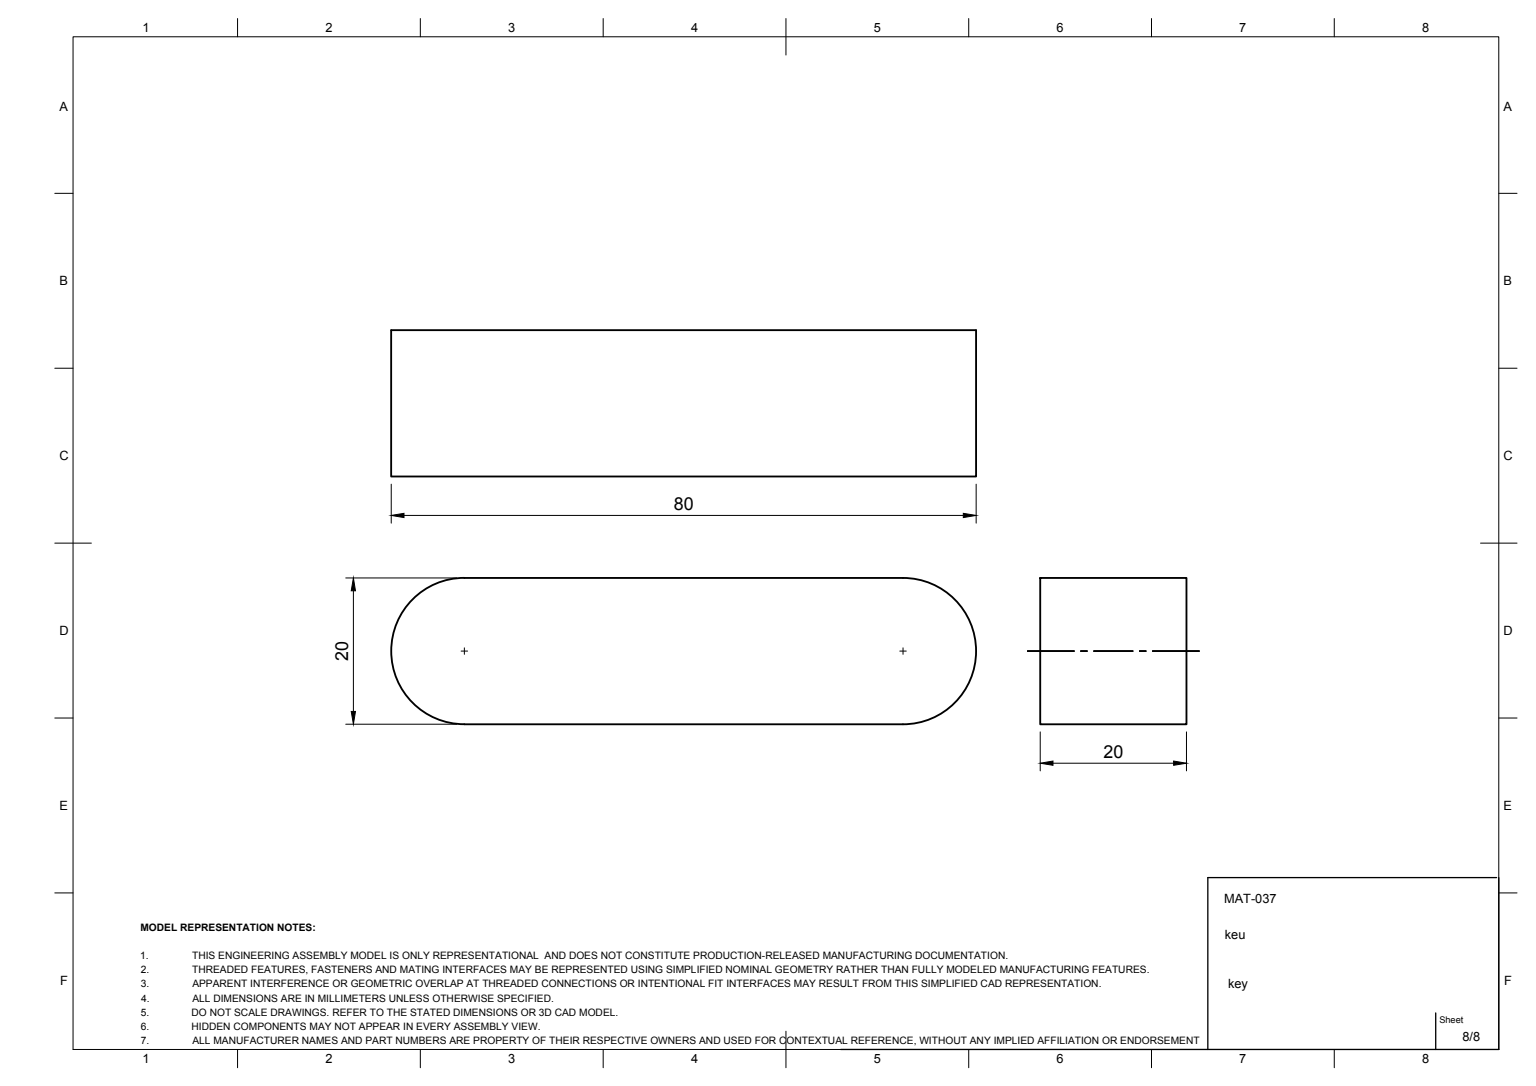
ISO-10303-21;
HEADER;
/* Generated by software containing ST-Developer
 * from STEP Tools, Inc. (www.steptools.com) 
 */

FILE_DESCRIPTION(
/* description */ ('STEP AP214'),
/* implementation_level */ '2;1');

FILE_NAME(
/* name */ 'key.step',
/* time_stamp */ '2026-11-14T21:09:07-08:00',
/* author */ (''),
/* organization */ (''),
/* preprocessor_version */ 'ST-DEVELOPER v20.2',
/* originating_system */ 'Autodesk Translation Framework v15.17.0.0',
/* authorisation */ '');

FILE_SCHEMA (('AUTOMOTIVE_DESIGN { 1 0 10303 214 3 1 1 }'));
ENDSEC;

DATA;
#10=MECHANICAL_DESIGN_GEOMETRIC_PRESENTATION_REPRESENTATION('',(#84),#2059);
#70=SHAPE_REPRESENTATION_RELATIONSHIP('SRR','None',#2100,#77);
#77=ADVANCED_BREP_SHAPE_REPRESENTATION('',(#91),#2058);
#84=STYLED_ITEM('',(#2141),#91);
#91=MANIFOLD_SOLID_BREP('Body1',#981);
#121=PLANE('',#1157);
#122=PLANE('',#1158);
#123=PLANE('',#1161);
#124=PLANE('',#1162);
#206=FACE_OUTER_BOUND('',#282,.T.);
#207=FACE_OUTER_BOUND('',#283,.T.);
#208=FACE_OUTER_BOUND('',#284,.T.);
#209=FACE_OUTER_BOUND('',#285,.T.);
#210=FACE_OUTER_BOUND('',#286,.T.);
#211=FACE_OUTER_BOUND('',#287,.T.);
#282=EDGE_LOOP('',(#873,#874,#875,#876));
#283=EDGE_LOOP('',(#877,#878,#879,#880));
#284=EDGE_LOOP('',(#881,#882,#883,#884));
#285=EDGE_LOOP('',(#885,#886,#887,#888));
#286=EDGE_LOOP('',(#889,#890,#891,#892));
#287=EDGE_LOOP('',(#893,#894,#895,#896));
#345=LINE('',#2006,#410);
#346=LINE('',#2008,#411);
#347=LINE('',#2010,#412);
#348=LINE('',#2011,#413);
#349=LINE('',#2016,#414);
#350=LINE('',#2020,#415);
#351=LINE('',#2022,#416);
#352=LINE('',#2023,#417);
#410=VECTOR('',#1433,1000.);
#411=VECTOR('',#1434,1000.);
#412=VECTOR('',#1435,1000.);
#413=VECTOR('',#1436,1000.);
#414=VECTOR('',#1441,1000.);
#415=VECTOR('',#1446,1000.);
#416=VECTOR('',#1447,1000.);
#417=VECTOR('',#1448,1000.);
#457=CIRCLE('',#1159,10.0000000000001);
#458=CIRCLE('',#1160,10.0000000000001);
#459=CIRCLE('',#1163,10.0000000000001);
#460=CIRCLE('',#1164,10.0000000000001);
#532=VERTEX_POINT('',#2004);
#533=VERTEX_POINT('',#2005);
#534=VERTEX_POINT('',#2007);
#535=VERTEX_POINT('',#2009);
#536=VERTEX_POINT('',#2013);
#537=VERTEX_POINT('',#2015);
#538=VERTEX_POINT('',#2019);
#539=VERTEX_POINT('',#2021);
#647=EDGE_CURVE('',#532,#533,#345,.T.);
#648=EDGE_CURVE('',#533,#534,#346,.T.);
#649=EDGE_CURVE('',#535,#534,#347,.T.);
#650=EDGE_CURVE('',#535,#532,#348,.T.);
#651=EDGE_CURVE('',#534,#536,#457,.T.);
#652=EDGE_CURVE('',#537,#536,#349,.T.);
#653=EDGE_CURVE('',#537,#535,#458,.T.);
#654=EDGE_CURVE('',#536,#538,#350,.T.);
#655=EDGE_CURVE('',#539,#538,#351,.T.);
#656=EDGE_CURVE('',#539,#537,#352,.T.);
#657=EDGE_CURVE('',#538,#533,#459,.T.);
#658=EDGE_CURVE('',#532,#539,#460,.T.);
#873=ORIENTED_EDGE('',*,*,#647,.T.);
#874=ORIENTED_EDGE('',*,*,#648,.T.);
#875=ORIENTED_EDGE('',*,*,#649,.F.);
#876=ORIENTED_EDGE('',*,*,#650,.T.);
#877=ORIENTED_EDGE('',*,*,#651,.T.);
#878=ORIENTED_EDGE('',*,*,#652,.F.);
#879=ORIENTED_EDGE('',*,*,#653,.T.);
#880=ORIENTED_EDGE('',*,*,#649,.T.);
#881=ORIENTED_EDGE('',*,*,#652,.T.);
#882=ORIENTED_EDGE('',*,*,#654,.T.);
#883=ORIENTED_EDGE('',*,*,#655,.F.);
#884=ORIENTED_EDGE('',*,*,#656,.T.);
#885=ORIENTED_EDGE('',*,*,#655,.T.);
#886=ORIENTED_EDGE('',*,*,#657,.T.);
#887=ORIENTED_EDGE('',*,*,#647,.F.);
#888=ORIENTED_EDGE('',*,*,#658,.T.);
#889=ORIENTED_EDGE('',*,*,#651,.F.);
#890=ORIENTED_EDGE('',*,*,#648,.F.);
#891=ORIENTED_EDGE('',*,*,#657,.F.);
#892=ORIENTED_EDGE('',*,*,#654,.F.);
#893=ORIENTED_EDGE('',*,*,#650,.F.);
#894=ORIENTED_EDGE('',*,*,#653,.F.);
#895=ORIENTED_EDGE('',*,*,#656,.F.);
#896=ORIENTED_EDGE('',*,*,#658,.F.);
#917=CYLINDRICAL_SURFACE('',#1165,10.0000000000001);
#918=CYLINDRICAL_SURFACE('',#1166,10.0000000000001);
#969=ADVANCED_FACE('',(#206),#121,.F.);
#970=ADVANCED_FACE('',(#207),#122,.F.);
#971=ADVANCED_FACE('',(#208),#123,.F.);
#972=ADVANCED_FACE('',(#209),#124,.F.);
#973=ADVANCED_FACE('',(#210),#917,.T.);
#974=ADVANCED_FACE('',(#211),#918,.T.);
#981=CLOSED_SHELL('',(#969,#970,#971,#972,#973,#974));
#1156=AXIS2_PLACEMENT_3D('',#2002,#1429,#1430);
#1157=AXIS2_PLACEMENT_3D('',#2003,#1431,#1432);
#1158=AXIS2_PLACEMENT_3D('',#2012,#1437,#1438);
#1159=AXIS2_PLACEMENT_3D('',#2014,#1439,#1440);
#1160=AXIS2_PLACEMENT_3D('',#2017,#1442,#1443);
#1161=AXIS2_PLACEMENT_3D('',#2018,#1444,#1445);
#1162=AXIS2_PLACEMENT_3D('',#2024,#1449,#1450);
#1163=AXIS2_PLACEMENT_3D('',#2025,#1451,#1452);
#1164=AXIS2_PLACEMENT_3D('',#2026,#1453,#1454);
#1165=AXIS2_PLACEMENT_3D('',#2027,#1455,#1456);
#1166=AXIS2_PLACEMENT_3D('',#2028,#1457,#1458);
#1429=DIRECTION('axis',(0.,0.,1.));
#1430=DIRECTION('refdir',(1.,0.,0.));
#1431=DIRECTION('center_axis',(1.,-3.57452597678267E-31,1.04083408558607E-17));
#1432=DIRECTION('ref_axis',(1.04083408558607E-17,1.47911419728938E-31,-1.));
#1433=DIRECTION('',(1.04083408558607E-17,1.47911419728938E-31,-1.));
#1434=DIRECTION('',(3.6977854932235E-31,-1.,0.));
#1435=DIRECTION('',(1.04083408558607E-17,1.47911419728938E-31,-1.));
#1436=DIRECTION('',(-3.6977854932235E-31,1.,0.));
#1437=DIRECTION('center_axis',(-3.69778549322349E-31,1.,1.47911419728938E-31));
#1438=DIRECTION('ref_axis',(-1.04083408558607E-17,-1.47911419728938E-31,
1.));
#1439=DIRECTION('center_axis',(3.69778549322349E-31,-1.,0.));
#1440=DIRECTION('ref_axis',(-5.46944702155759E-62,-2.02248418522701E-92,
1.));
#1441=DIRECTION('',(1.04083408558607E-17,1.47911419728938E-31,-1.));
#1442=DIRECTION('center_axis',(3.69778549322349E-31,-1.,0.));
#1443=DIRECTION('ref_axis',(-5.46944702155759E-62,-2.02248418522701E-92,
1.));
#1444=DIRECTION('center_axis',(-1.,3.57452597678267E-31,-1.04083408558607E-17));
#1445=DIRECTION('ref_axis',(-1.04083408558607E-17,-1.47911419728938E-31,
1.));
#1446=DIRECTION('',(-3.6977854932235E-31,1.,0.));
#1447=DIRECTION('',(1.04083408558607E-17,1.47911419728938E-31,-1.));
#1448=DIRECTION('',(3.6977854932235E-31,-1.,0.));
#1449=DIRECTION('center_axis',(3.69778549322349E-31,-1.,-1.47911419728938E-31));
#1450=DIRECTION('ref_axis',(1.04083408558607E-17,1.47911419728938E-31,-1.));
#1451=DIRECTION('center_axis',(-3.69778549322349E-31,1.,0.));
#1452=DIRECTION('ref_axis',(-4.16507106582027E-13,-1.54015393654351E-43,
-1.));
#1453=DIRECTION('center_axis',(-3.69778549322349E-31,1.,0.));
#1454=DIRECTION('ref_axis',(0.,0.,-1.));
#1455=DIRECTION('center_axis',(-3.69778549322349E-31,1.,0.));
#1456=DIRECTION('ref_axis',(1.66655918373688E-13,6.16257837322063E-44,-1.));
#1457=DIRECTION('center_axis',(3.69778549322349E-31,-1.,0.));
#1458=DIRECTION('ref_axis',(1.10899837782601E-13,4.1008381135334E-44,1.));
#2002=CARTESIAN_POINT('',(0.,0.,0.));
#2003=CARTESIAN_POINT('Origin',(9.99200722162641E-13,-1.11022302462516E-13,
80.0000000000001));
#2004=CARTESIAN_POINT('',(-5.55111512312578E-14,20.,70.0000000000016));
#2005=CARTESIAN_POINT('',(9.99200722162641E-13,20.,9.9999999999969));
#2006=CARTESIAN_POINT('',(9.99200722162641E-13,19.9999999999999,80.0000000000001));
#2007=CARTESIAN_POINT('',(9.99200722162641E-13,0.,9.9999999999969));
#2008=CARTESIAN_POINT('',(9.99200722162641E-13,0.,9.9999999999969));
#2009=CARTESIAN_POINT('',(-5.55111512312578E-14,0.,70.0000000000016));
#2010=CARTESIAN_POINT('',(9.99200722162641E-13,-1.11022302462516E-13,80.0000000000001));
#2011=CARTESIAN_POINT('',(-5.55111512312578E-14,0.,70.0000000000016));
#2012=CARTESIAN_POINT('Origin',(9.99200722162641E-13,-1.11022302462516E-13,
80.0000000000001));
#2013=CARTESIAN_POINT('',(20.0000000000001,0.,10.0000000000002));
#2014=CARTESIAN_POINT('Origin',(10.0000000000001,0.,10.0000000000002));
#2015=CARTESIAN_POINT('',(20.000000000001,-1.11022302462516E-13,69.9999999999994));
#2016=CARTESIAN_POINT('',(20.0000000000001,-1.11022302462516E-13,80.0000000000003));
#2017=CARTESIAN_POINT('Origin',(10.000000000001,0.,70.0000000000005));
#2018=CARTESIAN_POINT('Origin',(20.0000000000001,-1.11022302462516E-13,
80.0000000000003));
#2019=CARTESIAN_POINT('',(20.0000000000001,20.,10.0000000000002));
#2020=CARTESIAN_POINT('',(20.0000000000001,20.,10.0000000000002));
#2021=CARTESIAN_POINT('',(20.000000000001,19.9999999999999,69.9999999999994));
#2022=CARTESIAN_POINT('',(20.0000000000001,19.9999999999999,80.0000000000003));
#2023=CARTESIAN_POINT('',(20.000000000001,-1.11022302462516E-13,69.9999999999994));
#2024=CARTESIAN_POINT('Origin',(9.99200722162641E-13,19.9999999999999,80.0000000000001));
#2025=CARTESIAN_POINT('Origin',(10.0000000000001,20.,10.0000000000002));
#2026=CARTESIAN_POINT('Origin',(10.000000000001,20.,70.0000000000005));
#2027=CARTESIAN_POINT('Origin',(10.0000000000001,0.,10.0000000000002));
#2028=CARTESIAN_POINT('Origin',(10.000000000001,0.,70.0000000000005));
#2049=UNCERTAINTY_MEASURE_WITH_UNIT(LENGTH_MEASURE(0.01),#2060,
'DISTANCE_ACCURACY_VALUE',
'Maximum model space distance between geometric entities at asserted c
onnectivities');
#2050=UNCERTAINTY_MEASURE_WITH_UNIT(LENGTH_MEASURE(0.01),#2060,
'DISTANCE_ACCURACY_VALUE',
'Maximum model space distance between geometric entities at asserted c
onnectivities');
#2058=(
GEOMETRIC_REPRESENTATION_CONTEXT(3)
GLOBAL_UNCERTAINTY_ASSIGNED_CONTEXT((#2049))
GLOBAL_UNIT_ASSIGNED_CONTEXT((#2060,#2062,#2063))
REPRESENTATION_CONTEXT('','3D')
);
#2059=(
GEOMETRIC_REPRESENTATION_CONTEXT(3)
GLOBAL_UNCERTAINTY_ASSIGNED_CONTEXT((#2050))
GLOBAL_UNIT_ASSIGNED_CONTEXT((#2060,#2062,#2063))
REPRESENTATION_CONTEXT('','3D')
);
#2060=(
LENGTH_UNIT()
NAMED_UNIT(*)
SI_UNIT(.MILLI.,.METRE.)
);
#2062=(
NAMED_UNIT(*)
PLANE_ANGLE_UNIT()
SI_UNIT($,.RADIAN.)
);
#2063=(
NAMED_UNIT(*)
SI_UNIT($,.STERADIAN.)
SOLID_ANGLE_UNIT()
);
#2071=SHAPE_DEFINITION_REPRESENTATION(#2079,#2100);
#2079=PRODUCT_DEFINITION_SHAPE('',$,#2109);
#2100=SHAPE_REPRESENTATION('',(#1156),#2058);
#2101=PRODUCT_DEFINITION_CONTEXT('part definition',#2127,'design');
#2109=PRODUCT_DEFINITION('keu','key',#2117,#2101);
#2117=PRODUCT_DEFINITION_FORMATION('',$,#2136);
#2127=APPLICATION_CONTEXT(
'Core Data for Automotive Mechanical Design Process');
#2128=PRODUCT_CONTEXT('part definition',#2127,'mechanical');
#2136=PRODUCT('keu','key',$,(#2128));
#2141=PRESENTATION_STYLE_ASSIGNMENT((#2147));
#2147=SURFACE_STYLE_USAGE(.BOTH.,#2153);
#2153=SURFACE_SIDE_STYLE('',(#2159));
#2159=SURFACE_STYLE_FILL_AREA(#2165);
#2165=FILL_AREA_STYLE('Opaque(97,158,199)',(#2171));
#2171=FILL_AREA_STYLE_COLOUR('Opaque(97,158,199)',#2177);
#2177=COLOUR_RGB('Opaque(97,158,199)',0.380392156862745,0.619607843137255,
0.780392156862745);
ENDSEC;
END-ISO-10303-21;
